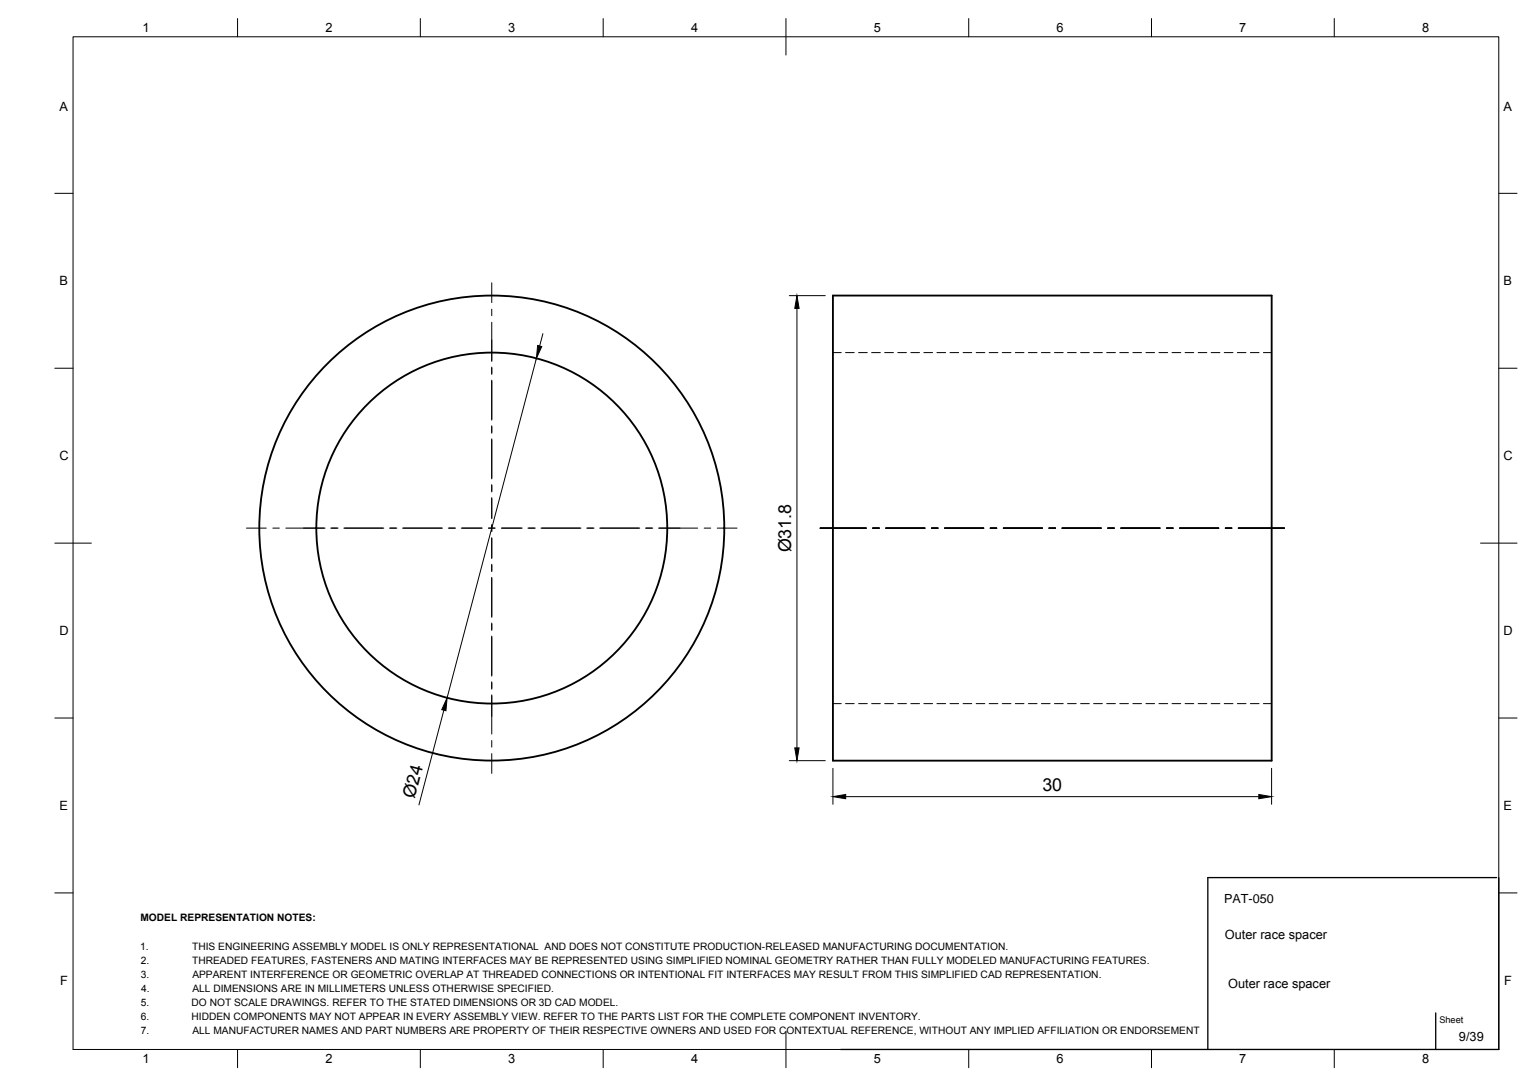
ISO-10303-21;
HEADER;
/* Generated by software containing ST-Developer
 * from STEP Tools, Inc. (www.steptools.com) 
 */

FILE_DESCRIPTION(
/* description */ ('Hand wheel with handle and shaft collar'),
/* implementation_level */ '2;1');

FILE_NAME(
/* name */ 'Outer race spacer.step',
/* time_stamp */ '2026-10-28T03:23:19-07:00',
/* author */ (''),
/* organization */ (''),
/* preprocessor_version */ 'ST-DEVELOPER v20.2',
/* originating_system */ 'Autodesk Translation Framework v15.17.0.0',
/* authorisation */ '');

FILE_SCHEMA (('AUTOMOTIVE_DESIGN { 1 0 10303 214 3 1 1 }'));
ENDSEC;

DATA;
#10=MECHANICAL_DESIGN_GEOMETRIC_PRESENTATION_REPRESENTATION('',(#399),#10510);
#335=SHAPE_REPRESENTATION_RELATIONSHIP('SRR','None',#10651,#367);
#367=ADVANCED_BREP_SHAPE_REPRESENTATION('',(#446),#10478);
#399=STYLED_ITEM('',(#10908),#446);
#446=MANIFOLD_SOLID_BREP('Body1',#5298);
#512=FACE_BOUND('',#1152,.T.);
#513=FACE_BOUND('',#1154,.T.);
#626=PLANE('',#5777);
#627=PLANE('',#5778);
#804=FACE_OUTER_BOUND('',#1149,.T.);
#805=FACE_OUTER_BOUND('',#1150,.T.);
#806=FACE_OUTER_BOUND('',#1151,.T.);
#807=FACE_OUTER_BOUND('',#1153,.T.);
#1149=EDGE_LOOP('',(#3755,#3756,#3757,#3758));
#1150=EDGE_LOOP('',(#3759,#3760,#3761,#3762));
#1151=EDGE_LOOP('',(#3763));
#1152=EDGE_LOOP('',(#3764));
#1153=EDGE_LOOP('',(#3765));
#1154=EDGE_LOOP('',(#3766));
#1586=LINE('',#8390,#1896);
#1587=LINE('',#8396,#1897);
#1896=VECTOR('',#6644,1.2);
#1897=VECTOR('',#6651,1.59);
#2159=CIRCLE('',#5772,1.2);
#2160=CIRCLE('',#5773,1.2);
#2161=CIRCLE('',#5775,1.59);
#2162=CIRCLE('',#5776,1.59);
#2510=VERTEX_POINT('',#8387);
#2511=VERTEX_POINT('',#8389);
#2512=VERTEX_POINT('',#8393);
#2513=VERTEX_POINT('',#8395);
#2995=EDGE_CURVE('',#2510,#2510,#2159,.T.);
#2996=EDGE_CURVE('',#2510,#2511,#1586,.T.);
#2997=EDGE_CURVE('',#2511,#2511,#2160,.T.);
#2998=EDGE_CURVE('',#2512,#2512,#2161,.T.);
#2999=EDGE_CURVE('',#2512,#2513,#1587,.T.);
#3000=EDGE_CURVE('',#2513,#2513,#2162,.T.);
#3755=ORIENTED_EDGE('',*,*,#2995,.F.);
#3756=ORIENTED_EDGE('',*,*,#2996,.T.);
#3757=ORIENTED_EDGE('',*,*,#2997,.T.);
#3758=ORIENTED_EDGE('',*,*,#2996,.F.);
#3759=ORIENTED_EDGE('',*,*,#2998,.F.);
#3760=ORIENTED_EDGE('',*,*,#2999,.T.);
#3761=ORIENTED_EDGE('',*,*,#3000,.T.);
#3762=ORIENTED_EDGE('',*,*,#2999,.F.);
#3763=ORIENTED_EDGE('',*,*,#2998,.T.);
#3764=ORIENTED_EDGE('',*,*,#2995,.T.);
#3765=ORIENTED_EDGE('',*,*,#3000,.F.);
#3766=ORIENTED_EDGE('',*,*,#2997,.F.);
#4892=CYLINDRICAL_SURFACE('',#5771,1.2);
#4893=CYLINDRICAL_SURFACE('',#5774,1.59);
#5016=ADVANCED_FACE('',(#804),#4892,.F.);
#5017=ADVANCED_FACE('',(#805),#4893,.T.);
#5018=ADVANCED_FACE('',(#806,#512),#626,.T.);
#5019=ADVANCED_FACE('',(#807,#513),#627,.F.);
#5298=CLOSED_SHELL('',(#5016,#5017,#5018,#5019));
#5770=AXIS2_PLACEMENT_3D('',#8385,#6638,#6639);
#5771=AXIS2_PLACEMENT_3D('',#8386,#6640,#6641);
#5772=AXIS2_PLACEMENT_3D('',#8388,#6642,#6643);
#5773=AXIS2_PLACEMENT_3D('',#8391,#6645,#6646);
#5774=AXIS2_PLACEMENT_3D('',#8392,#6647,#6648);
#5775=AXIS2_PLACEMENT_3D('',#8394,#6649,#6650);
#5776=AXIS2_PLACEMENT_3D('',#8397,#6652,#6653);
#5777=AXIS2_PLACEMENT_3D('',#8398,#6654,#6655);
#5778=AXIS2_PLACEMENT_3D('',#8399,#6656,#6657);
#6638=DIRECTION('axis',(0.,0.,1.));
#6639=DIRECTION('refdir',(1.,0.,0.));
#6640=DIRECTION('center_axis',(0.,1.,0.));
#6641=DIRECTION('ref_axis',(1.,0.,0.));
#6642=DIRECTION('center_axis',(0.,-1.,0.));
#6643=DIRECTION('ref_axis',(1.,0.,0.));
#6644=DIRECTION('',(0.,-1.,0.));
#6645=DIRECTION('center_axis',(0.,-1.,0.));
#6646=DIRECTION('ref_axis',(1.,0.,0.));
#6647=DIRECTION('center_axis',(0.,1.,0.));
#6648=DIRECTION('ref_axis',(1.,0.,0.));
#6649=DIRECTION('center_axis',(0.,1.,0.));
#6650=DIRECTION('ref_axis',(1.,0.,0.));
#6651=DIRECTION('',(0.,-1.,0.));
#6652=DIRECTION('center_axis',(0.,1.,0.));
#6653=DIRECTION('ref_axis',(1.,0.,0.));
#6654=DIRECTION('center_axis',(0.,1.,0.));
#6655=DIRECTION('ref_axis',(1.,0.,0.));
#6656=DIRECTION('center_axis',(0.,1.,0.));
#6657=DIRECTION('ref_axis',(1.,0.,0.));
#8385=CARTESIAN_POINT('',(0.,0.,0.));
#8386=CARTESIAN_POINT('Origin',(0.,0.5,10.));
#8387=CARTESIAN_POINT('',(-1.2,3.5,10.));
#8388=CARTESIAN_POINT('Origin',(0.,3.5,10.));
#8389=CARTESIAN_POINT('',(-1.2,0.5,10.));
#8390=CARTESIAN_POINT('',(-1.2,0.5,10.));
#8391=CARTESIAN_POINT('Origin',(0.,0.5,10.));
#8392=CARTESIAN_POINT('Origin',(0.,0.5,10.));
#8393=CARTESIAN_POINT('',(-1.59,3.5,10.));
#8394=CARTESIAN_POINT('Origin',(0.,3.5,10.));
#8395=CARTESIAN_POINT('',(-1.59,0.5,10.));
#8396=CARTESIAN_POINT('',(-1.59,0.5,10.));
#8397=CARTESIAN_POINT('Origin',(0.,0.5,10.));
#8398=CARTESIAN_POINT('Origin',(0.,3.5,10.));
#8399=CARTESIAN_POINT('Origin',(0.,0.5,10.));
#10439=UNCERTAINTY_MEASURE_WITH_UNIT(LENGTH_MEASURE(0.001),#10511,
'DISTANCE_ACCURACY_VALUE',
'Maximum model space distance between geometric entities at asserted c
onnectivities');
#10471=UNCERTAINTY_MEASURE_WITH_UNIT(LENGTH_MEASURE(0.001),#10511,
'DISTANCE_ACCURACY_VALUE',
'Maximum model space distance between geometric entities at asserted c
onnectivities');
#10478=(
GEOMETRIC_REPRESENTATION_CONTEXT(3)
GLOBAL_UNCERTAINTY_ASSIGNED_CONTEXT((#10439))
GLOBAL_UNIT_ASSIGNED_CONTEXT((#10511,#10513,#10514))
REPRESENTATION_CONTEXT('','3D')
);
#10510=(
GEOMETRIC_REPRESENTATION_CONTEXT(3)
GLOBAL_UNCERTAINTY_ASSIGNED_CONTEXT((#10471))
GLOBAL_UNIT_ASSIGNED_CONTEXT((#10511,#10513,#10514))
REPRESENTATION_CONTEXT('','3D')
);
#10511=(
LENGTH_UNIT()
NAMED_UNIT(*)
SI_UNIT(.CENTI.,.METRE.)
);
#10513=(
NAMED_UNIT(*)
PLANE_ANGLE_UNIT()
SI_UNIT($,.RADIAN.)
);
#10514=(
NAMED_UNIT(*)
SI_UNIT($,.STERADIAN.)
SOLID_ANGLE_UNIT()
);
#10521=SHAPE_DEFINITION_REPRESENTATION(#10559,#10651);
#10559=PRODUCT_DEFINITION_SHAPE('',$,#10690);
#10651=SHAPE_REPRESENTATION('',(#5770),#10478);
#10683=PRODUCT_DEFINITION_CONTEXT('part definition',#10799,'design');
#10690=PRODUCT_DEFINITION('Outer race spacer','Outer race spacer',#10728,
#10683);
#10728=PRODUCT_DEFINITION_FORMATION('',$,#10807);
#10799=APPLICATION_CONTEXT(
'Core Data for Automotive Mechanical Design Process');
#10800=PRODUCT_CONTEXT('part definition',#10799,'mechanical');
#10807=PRODUCT('Outer race spacer','Outer race spacer',
'Outer race spacer',(#10800));
#10902=COLOUR_RGB('Grey',0.48,0.52,0.57);
#10903=FILL_AREA_STYLE_COLOUR('',#10902);
#10904=FILL_AREA_STYLE('',(#10903));
#10905=SURFACE_STYLE_FILL_AREA(#10904);
#10906=SURFACE_SIDE_STYLE('',(#10905));
#10907=SURFACE_STYLE_USAGE(.BOTH.,#10906);
#10908=PRESENTATION_STYLE_ASSIGNMENT((#10907));
ENDSEC;
END-ISO-10303-21;
